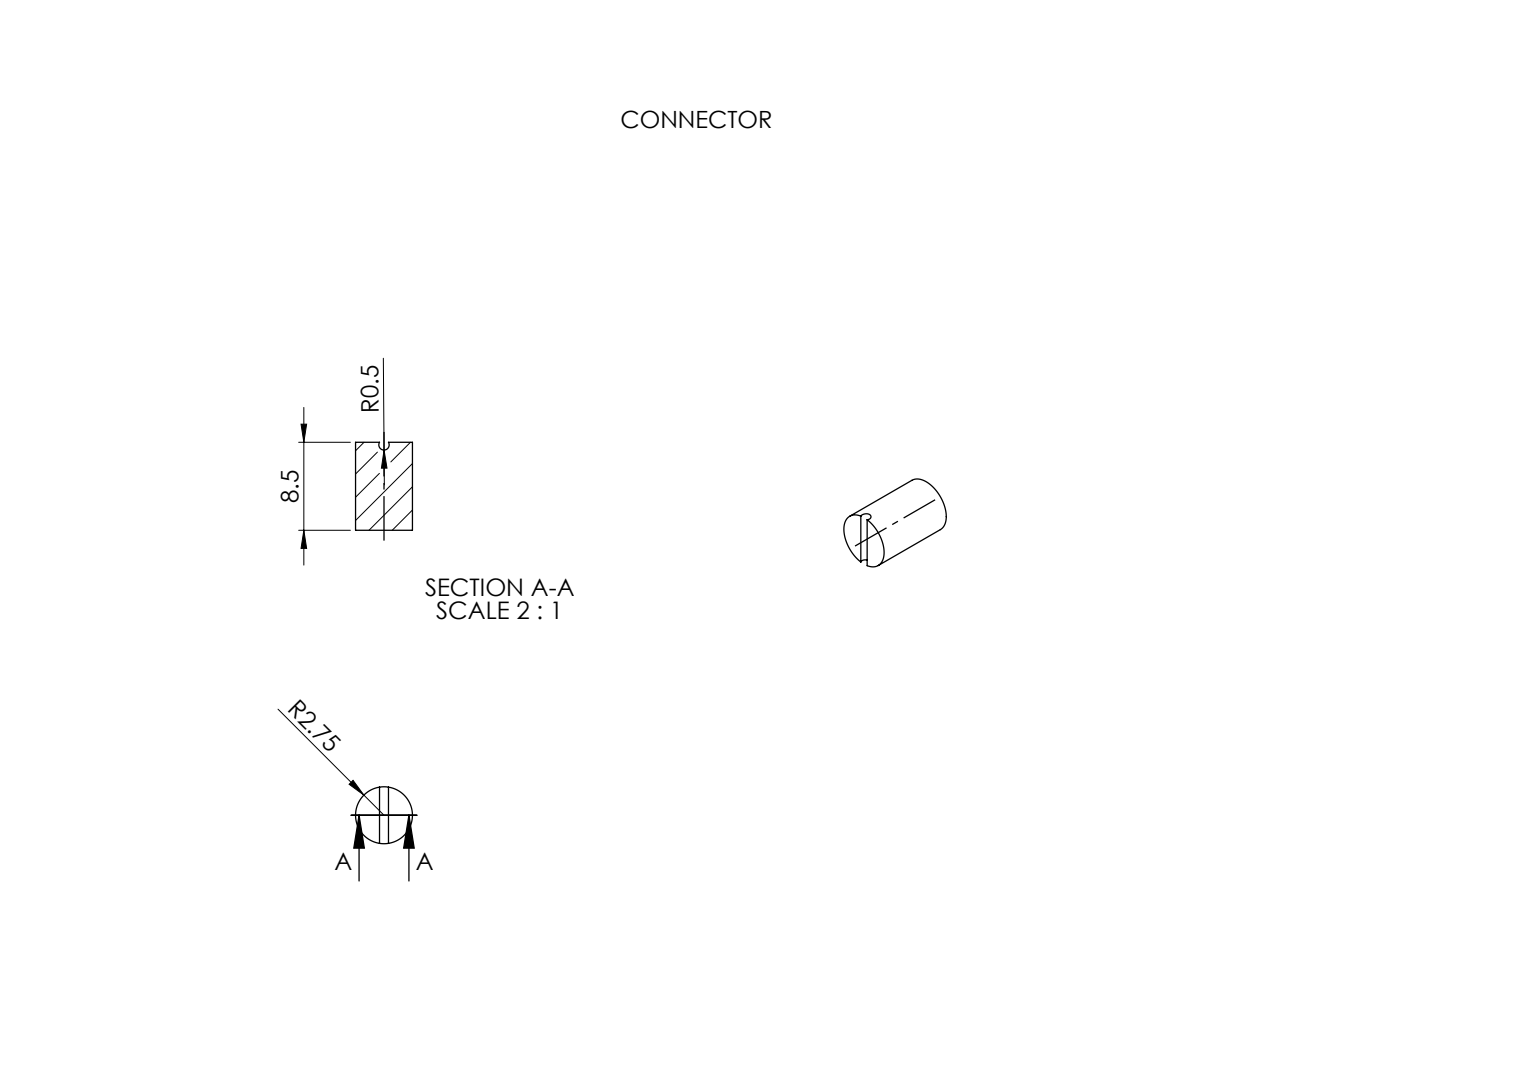
ISO-10303-21;
HEADER;
FILE_DESCRIPTION (('STEP AP214'),
    '1' );
FILE_NAME ('connector.step',
    '2026-10-05T05:16:24',
    ( '' ),
    ( '' ),
    'SwSTEP 2.0',
    'SolidWorks 2026',
    '' );
FILE_SCHEMA (( 'AUTOMOTIVE_DESIGN' ));
ENDSEC;

DATA;
#1351=DIRECTION ( 'NONE',  ( 1.000000000000000000, 0.000000000000000000, -0.000000000000000000 ) ) ;
#1835=( GEOMETRIC_REPRESENTATION_CONTEXT ( 3 ) GLOBAL_UNCERTAINTY_ASSIGNED_CONTEXT ( ( #35290 ) ) GLOBAL_UNIT_ASSIGNED_CONTEXT ( ( #39286, #45578, #18562 ) ) REPRESENTATION_CONTEXT ( 'NONE', 'WORKASPACE' ) );
#2791=VERTEX_POINT ( 'NONE', #87496 ) ;
#2984=PRODUCT_DEFINITION_FORMATION_WITH_SPECIFIED_SOURCE ( 'ANY', '', #6674, .NOT_KNOWN. ) ;
#3686=EDGE_LOOP ( 'NONE', ( #46969, #18682, #79831, #72227, #6479, #3837 ) ) ;
#3837=ORIENTED_EDGE ( 'NONE', *, *, #29448, .T. ) ;
#3884=AXIS2_PLACEMENT_3D ( 'NONE', #41339, #8443, #62915 ) ;
#3912=CARTESIAN_POINT ( 'NONE',  ( 0.4769952865663710795, -10.20868217879685425, 29.42381992869616880 ) ) ;
#4377=CARTESIAN_POINT ( 'NONE',  ( -0.1741240272142571821, -4.754468449490619086, 28.77324492963870028 ) ) ;
#4547=DIRECTION ( 'NONE',  ( -0.000000000000000000, -1.000000000000000000, -0.000000000000000000 ) ) ;
#4578=SHAPE_DEFINITION_REPRESENTATION ( #68530, #14956 ) ;
#4670=AXIS2_PLACEMENT_3D ( 'NONE', #7512, #21903, #77287 ) ;
#4814=EDGE_CURVE ( 'NONE', #33014, #88650, #15467, .T. ) ;
#5219=ADVANCED_FACE ( 'NONE', ( #76095 ), #23689, .F. ) ;
#5480=CARTESIAN_POINT ( 'NONE',  ( 1.653273178848927064E-15, -7.500000000000000000, 29.50000000000000355 ) ) ;
#5710=CARTESIAN_POINT ( 'NONE',  ( -0.4998584449498338911, -4.795810369898659609, 29.16127627612525330 ) ) ;
#6479=ORIENTED_EDGE ( 'NONE', *, *, #71103, .T. ) ;
#6620=VECTOR ( 'NONE', #30863, 1000.000000000000000 ) ;
#6674=PRODUCT ( 'connector', 'connector', '', ( #46889 ) ) ;
#7417=CARTESIAN_POINT ( 'NONE',  ( 1.653273178848927064E-15, -7.500000000000000000, 29.50000000000000355 ) ) ;
#7512=CARTESIAN_POINT ( 'NONE',  ( 1.653273178848927064E-15, -7.500000000000000000, 21.00000000000000000 ) ) ;
#8399=APPLICATION_CONTEXT ( 'automotive_design' ) ;
#8443=DIRECTION ( 'NONE',  ( -0.000000000000000000, -0.000000000000000000, -1.000000000000000000 ) ) ;
#8469=DIRECTION ( 'NONE',  ( -1.000000000000000000, 0.000000000000000000, 0.000000000000000000 ) ) ;
#9364=CARTESIAN_POINT ( 'NONE',  ( -0.08744816603778379771, -10.24999508951804650, 28.75002700765198327 ) ) ;
#9375=VERTEX_POINT ( 'NONE', #63176 ) ;
#9793=CARTESIAN_POINT ( 'NONE',  ( 0.08713905105068281420, -10.25000490179539980, 28.74997304012405408 ) ) ;
#10109=EDGE_CURVE ( 'NONE', #88311, #16692, #87365, .T. ) ;
#10152=( GEOMETRIC_REPRESENTATION_CONTEXT ( 3 ) GLOBAL_UNCERTAINTY_ASSIGNED_CONTEXT ( ( #28487 ) ) GLOBAL_UNIT_ASSIGNED_CONTEXT ( ( #73982, #12270, #74417 ) ) REPRESENTATION_CONTEXT ( 'NONE', 'WORKASPACE' ) );
#10246=CARTESIAN_POINT ( 'NONE',  ( 0.3253212748352863892, -10.23174463298371073, 28.86040964833806299 ) ) ;
#10687=CARTESIAN_POINT ( 'NONE',  ( -0.4769917816027518520, -10.20868273765699819, 29.42382599947123722 ) ) ;
#11149=DIRECTION ( 'NONE',  ( 0.000000000000000000, 0.000000000000000000, 1.000000000000000000 ) ) ;
#11285=EDGE_CURVE ( 'NONE', #16692, #40474, #43288, .T. ) ;
#12141=CARTESIAN_POINT ( 'NONE',  ( -0.4330127018922180770, -4.750000000000000000, 29.50000000000000355 ) ) ;
#12270=( NAMED_UNIT ( * ) PLANE_ANGLE_UNIT ( ) SI_UNIT ( $, .RADIAN. ) );
#13472=AXIS2_PLACEMENT_3D ( 'NONE', #74758, #27007, #74309 ) ;
#13686=EDGE_CURVE ( 'NONE', #40474, #88311, #34853, .T. ) ;
#14956=SHAPE_REPRESENTATION ( 'connector', ( #83448 ), #41778 ) ;
#14978=UNCERTAINTY_MEASURE_WITH_UNIT (LENGTH_MEASURE( 1.000000000000000082E-05 ), #26230, 'distance_accuracy_value', 'NONE');
#15253=DIRECTION ( 'NONE',  ( 1.000000000000000000, 0.000000000000000000, 0.000000000000000000 ) ) ;
#15467=CIRCLE ( 'NONE', #29797, 2.750000000000000000 ) ;
#16165=COLOUR_RGB ( '', 0.40784314, 0.44705882, 0.49803922) ;
#16692=VERTEX_POINT ( 'NONE', #79353 ) ;
#16815=EDGE_CURVE ( 'NONE', #33014, #76058, #27958, .T. ) ;
#17033=ADVANCED_BREP_SHAPE_REPRESENTATION ( '', ( #28008, #83448 ), #41778 ) ;
#17628=CARTESIAN_POINT ( 'NONE',  ( 0.4330127018922180770, -4.750000000000000000, 29.50000000000000355 ) ) ;
#17974=ORIENTED_EDGE ( 'NONE', *, *, #29448, .F. ) ;
#18120=SURFACE_SIDE_STYLE ('',( #54548 ) ) ;
#18186=ORIENTED_EDGE ( 'NONE', *, *, #10109, .T. ) ;
#18562=( NAMED_UNIT ( * ) SI_UNIT ( $, .STERADIAN. ) SOLID_ANGLE_UNIT ( ) );
#18682=ORIENTED_EDGE ( 'NONE', *, *, #62994, .F. ) ;
#18955=LINE ( 'NONE', #17628, #42535 ) ;
#19445=SURFACE_STYLE_USAGE ( .BOTH. , #18120 ) ;
#19470=SURFACE_STYLE_FILL_AREA ( #74872 ) ;
#19666=CARTESIAN_POINT ( 'NONE',  ( -0.4330127018922180770, -4.784304877199946127, 29.50000000000000355 ) ) ;
#20322=CARTESIAN_POINT ( 'NONE',  ( -2.749999999999998224, -7.500000000000000000, 29.50000000000000355 ) ) ;
#20344=EDGE_CURVE ( 'NONE', #88650, #2791, #18955, .T. ) ;
#20368=SURFACE_SIDE_STYLE ('',( #19470 ) ) ;
#21810=DIRECTION ( 'NONE',  ( 0.000000000000000000, 0.000000000000000000, 1.000000000000000000 ) ) ;
#21903=DIRECTION ( 'NONE',  ( 0.000000000000000000, 0.000000000000000000, 1.000000000000000000 ) ) ;
#22045=DIRECTION ( 'NONE',  ( 0.000000000000000000, 0.000000000000000000, 1.000000000000000000 ) ) ;
#23689=CYLINDRICAL_SURFACE ( 'NONE', #54266, 0.5000000000000004441 ) ;
#23834=CARTESIAN_POINT ( 'NONE',  ( 1.653273178848927064E-15, -7.500000000000000000, 29.50000000000000355 ) ) ;
#23893=FACE_OUTER_BOUND ( 'NONE', #86429, .T. ) ;
#24639=CARTESIAN_POINT ( 'NONE',  ( 0.3892027609374598685, -10.22267510014235370, 28.92434864502809688 ) ) ;
#24662=FACE_OUTER_BOUND ( 'NONE', #63547, .T. ) ;
#24786=AXIS2_PLACEMENT_3D ( 'NONE', #72092, #65331, #52265 ) ;
#25084=CARTESIAN_POINT ( 'NONE',  ( -0.4330127018922180770, -10.21569512280005299, 29.50000000000000355 ) ) ;
#25379=PRODUCT_DEFINITION ( 'UNKNOWN', '', #2984, #30258 ) ;
#25540=CARTESIAN_POINT ( 'NONE',  ( 0.4765651934480724106, -4.791246328801548771, 29.07531184057632601 ) ) ;
#26230=( LENGTH_UNIT ( ) NAMED_UNIT ( * ) SI_UNIT ( .MILLI., .METRE. ) );
#26433=CARTESIAN_POINT ( 'NONE',  ( -0.08713905105068302237, -4.749995098204598420, 28.74997304012405763 ) ) ;
#26982=DIRECTION ( 'NONE',  ( 0.000000000000000000, 1.000000000000000000, 0.000000000000000000 ) ) ;
#27007=DIRECTION ( 'NONE',  ( 0.000000000000000000, 0.000000000000000000, 1.000000000000000000 ) ) ;
#27623=ORIENTED_EDGE ( 'NONE', *, *, #4814, .T. ) ;
#27675=STYLED_ITEM ( 'NONE', ( #67197 ), #28008 ) ;
#27958=LINE ( 'NONE', #35154, #29073 ) ;
#28008=MANIFOLD_SOLID_BREP ( 'Cut-Extrude2', #84621 ) ;
#28487=UNCERTAINTY_MEASURE_WITH_UNIT (LENGTH_MEASURE( 1.000000000000000082E-05 ), #73982, 'distance_accuracy_value', 'NONE');
#29073=VECTOR ( 'NONE', #62180, 1000.000000000000000 ) ;
#29332=DIRECTION ( 'NONE',  ( 1.000000000000000000, 0.000000000000000000, 0.000000000000000000 ) ) ;
#29351=ORIENTED_EDGE ( 'NONE', *, *, #4814, .F. ) ;
#29448=EDGE_CURVE ( 'NONE', #9375, #76058, #45082, .T. ) ;
#29797=AXIS2_PLACEMENT_3D ( 'NONE', #7417, #21810, #83528 ) ;
#30070=CARTESIAN_POINT ( 'NONE',  ( 0.4330127018922180770, -10.21569512280005299, 29.50000000000000355 ) ) ;
#30089=DIRECTION ( 'NONE',  ( 0.000000000000000000, 0.000000000000000000, 1.000000000000000000 ) ) ;
#30129=ORIENTED_EDGE ( 'NONE', *, *, #68190, .T. ) ;
#30258=PRODUCT_DEFINITION_CONTEXT ( 'detailed design', #8399, 'design' ) ;
#30863=DIRECTION ( 'NONE',  ( -0.000000000000000000, -0.000000000000000000, -1.000000000000000000 ) ) ;
#31502=DIRECTION ( 'NONE',  ( 1.000000000000000000, 0.000000000000000000, 0.000000000000000000 ) ) ;
#31859=CARTESIAN_POINT ( 'NONE',  ( 0.3256479613346660584, -4.768304711466844203, 28.86076157308317391 ) ) ;
#32650=CARTESIAN_POINT ( 'NONE',  ( -2.749999999999998224, -7.500000000000000000, 29.50000000000000355 ) ) ;
#32990=SURFACE_STYLE_USAGE ( .BOTH. , #20368 ) ;
#33014=VERTEX_POINT ( 'NONE', #70463 ) ;
#33986=ORIENTED_EDGE ( 'NONE', *, *, #11285, .T. ) ;
#34580=FACE_OUTER_BOUND ( 'NONE', #40204, .T. ) ;
#34853=CIRCLE ( 'NONE', #85196, 2.750000000000000000 ) ;
#35154=CARTESIAN_POINT ( 'NONE',  ( 2.750000000000001776, -7.500000000000000000, 29.50000000000000355 ) ) ;
#35290=UNCERTAINTY_MEASURE_WITH_UNIT (LENGTH_MEASURE( 1.000000000000000082E-05 ), #39286, 'distance_accuracy_value', 'NONE');
#35307=DIRECTION ( 'NONE',  ( 1.000000000000000000, 0.000000000000000000, 0.000000000000000000 ) ) ;
#35668=ORIENTED_EDGE ( 'NONE', *, *, #20344, .F. ) ;
#36822=CARTESIAN_POINT ( 'NONE',  ( 0.1741240272142571821, -10.24553155050938358, 28.77324492963869673 ) ) ;
#38152=CARTESIAN_POINT ( 'NONE',  ( -0.4765651934480722995, -10.20875367119844590, 29.07531184057631890 ) ) ;
#38624=DIRECTION ( 'NONE',  ( 1.000000000000000000, 0.000000000000000000, -0.000000000000000000 ) ) ;
#38763=PLANE ( 'NONE',  #24786 ) ;
#38891=MECHANICAL_DESIGN_GEOMETRIC_PRESENTATION_REPRESENTATION('',(#48969),#10152);
#39286=( LENGTH_UNIT ( ) NAMED_UNIT ( * ) SI_UNIT ( .MILLI., .METRE. ) );
#39512=CARTESIAN_POINT ( 'NONE',  ( -0.5001402707344744236, -4.795862479435460735, 29.33712102935293231 ) ) ;
#40204=EDGE_LOOP ( 'NONE', ( #29351, #45286, #68695, #61350, #40527, #61016 ) ) ;
#40398=CARTESIAN_POINT ( 'NONE',  ( 0.3891064303782384992, -4.777307027835201225, 28.92407589458995432 ) ) ;
#40474=VERTEX_POINT ( 'NONE', #20322 ) ;
#40527=ORIENTED_EDGE ( 'NONE', *, *, #11285, .F. ) ;
#41339=CARTESIAN_POINT ( 'NONE',  ( 1.653273178848927064E-15, -7.500000000000000000, 29.50000000000000355 ) ) ;
#41751=B_SPLINE_CURVE_WITH_KNOTS ( 'NONE', 3,
 ( #52111, #79600, #87260, #87707, #25540, #40398, #31859, #80040, #75067, #26433, #4377, #67856, #66066, #73744, #5710, #39512, #46254, #19666 ),
 .UNSPECIFIED., .F., .F.,
 ( 4, 2, 2, 2, 2, 2, 2, 2, 4 ),
 ( 0.000000000000000000, 0.0002610006692907291767, 0.0005220013385814583533, 0.0007830020078721875842, 0.001044002677162916707, 0.001305003346453645829, 0.001566004015744375168, 0.001827004685035104291, 0.002088005354325833413 ),
 .UNSPECIFIED. ) ;
#41778=( GEOMETRIC_REPRESENTATION_CONTEXT ( 3 ) GLOBAL_UNCERTAINTY_ASSIGNED_CONTEXT ( ( #14978 ) ) GLOBAL_UNIT_ASSIGNED_CONTEXT ( ( #26230, #60453, #87970 ) ) REPRESENTATION_CONTEXT ( 'NONE', 'WORKASPACE' ) );
#41884=CARTESIAN_POINT ( 'NONE',  ( 0.000000000000000000, -4.750000000000000000, 29.25000000000000000 ) ) ;
#42535=VECTOR ( 'NONE', #4547, 1000.000000000000000 ) ;
#42552=EDGE_CURVE ( 'NONE', #88650, #16692, #41751, .T. ) ;
#43038=ORIENTED_EDGE ( 'NONE', *, *, #55374, .F. ) ;
#43288=CIRCLE ( 'NONE', #79214, 2.750000000000000000 ) ;
#44818=LINE ( 'NONE', #32650, #6620 ) ;
#45082=CIRCLE ( 'NONE', #13472, 2.750000000000000000 ) ;
#45286=ORIENTED_EDGE ( 'NONE', *, *, #16815, .T. ) ;
#45346=CARTESIAN_POINT ( 'NONE',  ( -0.3891064303782384992, -10.22269297216479877, 28.92407589458995432 ) ) ;
#45578=( NAMED_UNIT ( * ) PLANE_ANGLE_UNIT ( ) SI_UNIT ( $, .RADIAN. ) );
#46254=CARTESIAN_POINT ( 'NONE',  ( -0.4769952865663709130, -4.791317821203144867, 29.42381992869616880 ) ) ;
#46889=PRODUCT_CONTEXT ( 'NONE', #82604, 'mechanical' ) ;
#46969=ORIENTED_EDGE ( 'NONE', *, *, #16815, .F. ) ;
#47379=SHAPE_REPRESENTATION_RELATIONSHIP ( 'NONE' , 'NONE' ,  #14956, #17033 ) ;
#48107=CYLINDRICAL_SURFACE ( 'NONE', #79255, 2.750000000000000000 ) ;
#48969=STYLED_ITEM ( 'NONE', ( #88841 ), #17033 ) ;
#50513=ORIENTED_EDGE ( 'NONE', *, *, #20344, .T. ) ;
#51640=CARTESIAN_POINT ( 'NONE',  ( -0.1752029071980582831, -10.24545254656222149, 28.77370482994317058 ) ) ;
#52111=CARTESIAN_POINT ( 'NONE',  ( 0.4330127018922180770, -4.784304877199946127, 29.50000000000000355 ) ) ;
#52126=PLANE ( 'NONE',  #54565 ) ;
#52265=DIRECTION ( 'NONE',  ( 1.000000000000000000, 0.000000000000000000, -0.000000000000000000 ) ) ;
#53068=ADVANCED_FACE ( 'NONE', ( #83695 ), #48107, .T. ) ;
#53177=ORIENTED_EDGE ( 'NONE', *, *, #62994, .T. ) ;
#53488=EDGE_LOOP ( 'NONE', ( #30129, #35668, #71447, #76985 ) ) ;
#53522=CIRCLE ( 'NONE', #4670, 2.750000000000000000 ) ;
#54266=AXIS2_PLACEMENT_3D ( 'NONE', #41884, #69786, #22045 ) ;
#54548=SURFACE_STYLE_FILL_AREA ( #61299 ) ;
#54565=AXIS2_PLACEMENT_3D ( 'NONE', #79614, #11149, #38624 ) ;
#55374=EDGE_CURVE ( 'NONE', #76058, #9375, #53522, .T. ) ;
#55410=CARTESIAN_POINT ( 'NONE',  ( 1.653273178848927064E-15, -7.500000000000000000, 29.50000000000000355 ) ) ;
#57551=ADVANCED_FACE ( 'NONE', ( #23893 ), #38763, .F. ) ;
#57975=CARTESIAN_POINT ( 'NONE',  ( -0.5000075107691263065, -10.20416206785629498, 29.33696104038924446 ) ) ;
#59725=CARTESIAN_POINT ( 'NONE',  ( 2.750000000000001776, -7.500000000000000000, 21.00000000000000000 ) ) ;
#60453=( NAMED_UNIT ( * ) PLANE_ANGLE_UNIT ( ) SI_UNIT ( $, .RADIAN. ) );
#61016=ORIENTED_EDGE ( 'NONE', *, *, #42552, .F. ) ;
#61299=FILL_AREA_STYLE ('',( #81160 ) ) ;
#61350=ORIENTED_EDGE ( 'NONE', *, *, #71103, .F. ) ;
#61893=COLOUR_RGB ( '', 0.40784314, 0.44705882, 0.49803922) ;
#62180=DIRECTION ( 'NONE',  ( -0.000000000000000000, -0.000000000000000000, -1.000000000000000000 ) ) ;
#62206=MECHANICAL_DESIGN_GEOMETRIC_PRESENTATION_REPRESENTATION('',(#27675),#1835);
#62763=CARTESIAN_POINT ( 'NONE',  ( 0.000000000000000000, 0.000000000000000000, 0.000000000000000000 ) ) ;
#62915=DIRECTION ( 'NONE',  ( -1.000000000000000000, 0.000000000000000000, 0.000000000000000000 ) ) ;
#62994=EDGE_CURVE ( 'NONE', #2791, #33014, #70001, .T. ) ;
#63176=CARTESIAN_POINT ( 'NONE',  ( -2.749999999999998224, -7.500000000000000000, 21.00000000000000000 ) ) ;
#63542=DIRECTION ( 'NONE',  ( 0.000000000000000000, 0.000000000000000000, 1.000000000000000000 ) ) ;
#63547=EDGE_LOOP ( 'NONE', ( #33986, #76979, #18186 ) ) ;
#64723=CARTESIAN_POINT ( 'NONE',  ( 0.4761625575576028391, -10.20882035374011565, 29.07450979259063928 ) ) ;
#65031=EDGE_LOOP ( 'NONE', ( #53177, #27623, #50513 ) ) ;
#65331=DIRECTION ( 'NONE',  ( 0.000000000000000000, 0.000000000000000000, 1.000000000000000000 ) ) ;
#66059=CARTESIAN_POINT ( 'NONE',  ( 0.5001402707344744236, -10.20413752056454193, 29.33712102935293942 ) ) ;
#66066=CARTESIAN_POINT ( 'NONE',  ( -0.3892027609374598685, -4.777324899857646301, 28.92434864502810399 ) ) ;
#66807=ADVANCED_FACE ( 'NONE', ( #77021 ), #70257, .T. ) ;
#67197=PRESENTATION_STYLE_ASSIGNMENT (( #19445 ) ) ;
#67856=CARTESIAN_POINT ( 'NONE',  ( -0.3253212748352862782, -4.768255367016290158, 28.86040964833806299 ) ) ;
#68190=EDGE_CURVE ( 'NONE', #88311, #2791, #83175, .T. ) ;
#68530=PRODUCT_DEFINITION_SHAPE ( 'NONE', 'NONE',  #25379 ) ;
#68695=ORIENTED_EDGE ( 'NONE', *, *, #55374, .T. ) ;
#69786=DIRECTION ( 'NONE',  ( 0.000000000000000000, 1.000000000000000000, 0.000000000000000000 ) ) ;
#69812=DIRECTION ( 'NONE',  ( 0.000000000000000000, 0.000000000000000000, 1.000000000000000000 ) ) ;
#70001=CIRCLE ( 'NONE', #78617, 2.750000000000000000 ) ;
#70158=DIRECTION ( 'NONE',  ( -0.000000000000000000, -0.000000000000000000, -1.000000000000000000 ) ) ;
#70257=PLANE ( 'NONE',  #73946 ) ;
#70463=CARTESIAN_POINT ( 'NONE',  ( 2.750000000000001776, -7.500000000000000000, 29.50000000000000355 ) ) ;
#70474=VECTOR ( 'NONE', #26982, 1000.000000000000000 ) ;
#71050=CARTESIAN_POINT ( 'NONE',  ( -0.4999924855028897164, -10.20416484602898954, 29.16295261168903252 ) ) ;
#71103=EDGE_CURVE ( 'NONE', #40474, #9375, #44818, .T. ) ;
#71447=ORIENTED_EDGE ( 'NONE', *, *, #42552, .T. ) ;
#71935=CARTESIAN_POINT ( 'NONE',  ( -0.3256479613346683899, -10.23169528853315491, 28.86076157308317391 ) ) ;
#72092=CARTESIAN_POINT ( 'NONE',  ( 1.653273178848927064E-15, -7.500000000000000000, 21.00000000000000000 ) ) ;
#72227=ORIENTED_EDGE ( 'NONE', *, *, #13686, .F. ) ;
#73744=CARTESIAN_POINT ( 'NONE',  ( -0.4761625575576027836, -4.791179646259885239, 29.07450979259064638 ) ) ;
#73946=AXIS2_PLACEMENT_3D ( 'NONE', #55410, #69812, #1351 ) ;
#73982=( LENGTH_UNIT ( ) NAMED_UNIT ( * ) SI_UNIT ( .MILLI., .METRE. ) );
#74309=DIRECTION ( 'NONE',  ( 1.000000000000000000, 0.000000000000000000, 0.000000000000000000 ) ) ;
#74417=( NAMED_UNIT ( * ) SI_UNIT ( $, .STERADIAN. ) SOLID_ANGLE_UNIT ( ) );
#74758=CARTESIAN_POINT ( 'NONE',  ( 1.653273178848927064E-15, -7.500000000000000000, 21.00000000000000000 ) ) ;
#74872=FILL_AREA_STYLE ('',( #81624 ) ) ;
#75067=CARTESIAN_POINT ( 'NONE',  ( 0.08744816603778360342, -4.750004910481952614, 28.75002700765199037 ) ) ;
#75557=CYLINDRICAL_SURFACE ( 'NONE', #3884, 2.750000000000000000 ) ;
#75889=ADVANCED_FACE ( 'NONE', ( #34580 ), #75557, .T. ) ;
#76058=VERTEX_POINT ( 'NONE', #59725 ) ;
#76095=FACE_OUTER_BOUND ( 'NONE', #53488, .T. ) ;
#76949=CARTESIAN_POINT ( 'NONE',  ( 1.653273178848927064E-15, -7.500000000000000000, 29.50000000000000355 ) ) ;
#76979=ORIENTED_EDGE ( 'NONE', *, *, #13686, .T. ) ;
#76985=ORIENTED_EDGE ( 'NONE', *, *, #10109, .F. ) ;
#77021=FACE_OUTER_BOUND ( 'NONE', #65031, .T. ) ;
#77287=DIRECTION ( 'NONE',  ( 1.000000000000000000, 0.000000000000000000, 0.000000000000000000 ) ) ;
#77948=CARTESIAN_POINT ( 'NONE',  ( 1.653273178848927064E-15, -7.500000000000000000, 29.50000000000000355 ) ) ;
#78617=AXIS2_PLACEMENT_3D ( 'NONE', #23834, #86006, #31502 ) ;
#79214=AXIS2_PLACEMENT_3D ( 'NONE', #76949, #30089, #15253 ) ;
#79255=AXIS2_PLACEMENT_3D ( 'NONE', #5480, #70158, #8469 ) ;
#79353=CARTESIAN_POINT ( 'NONE',  ( -0.4330127018922180770, -4.784304877199946127, 29.50000000000000355 ) ) ;
#79600=CARTESIAN_POINT ( 'NONE',  ( 0.4769917816027516855, -4.791317262343001815, 29.42382599947123722 ) ) ;
#79614=CARTESIAN_POINT ( 'NONE',  ( 1.653273178848927064E-15, -7.500000000000000000, 29.50000000000000355 ) ) ;
#79831=ORIENTED_EDGE ( 'NONE', *, *, #68190, .F. ) ;
#80040=CARTESIAN_POINT ( 'NONE',  ( 0.1752029071980549801, -4.754547453437774074, 28.77370482994318124 ) ) ;
#81160=FILL_AREA_STYLE_COLOUR ( '', #16165 ) ;
#81624=FILL_AREA_STYLE_COLOUR ( '', #61893 ) ;
#82604=APPLICATION_CONTEXT ( 'automotive_design' ) ;
#83175=B_SPLINE_CURVE_WITH_KNOTS ( 'NONE', 3,
 ( #25084, #10687, #57975, #71050, #38152, #45346, #71935, #51640, #9364, #9793, #36822, #10246, #24639, #64723, #85902, #66059, #3912, #30070 ),
 .UNSPECIFIED., .F., .F.,
 ( 4, 2, 2, 2, 2, 2, 2, 2, 4 ),
 ( 0.000000000000000000, 0.0002610006692907291224, 0.0005220013385814582449, 0.0007830020078721873673, 0.001044002677162916490, 0.001305003346453645612, 0.001566004015744375168, 0.001827004685035104291, 0.002088005354325833847 ),
 .UNSPECIFIED. ) ;
#83448=AXIS2_PLACEMENT_3D ( 'NONE', #62763, #83959, #35307 ) ;
#83528=DIRECTION ( 'NONE',  ( 1.000000000000000000, 0.000000000000000000, 0.000000000000000000 ) ) ;
#83695=FACE_OUTER_BOUND ( 'NONE', #3686, .T. ) ;
#83959=DIRECTION ( 'NONE',  ( 0.000000000000000000, 0.000000000000000000, 1.000000000000000000 ) ) ;
#84382=CARTESIAN_POINT ( 'NONE',  ( -0.4330127018922180770, -10.21569512280005299, 29.50000000000000355 ) ) ;
#84621=CLOSED_SHELL ( 'NONE', ( #75889, #53068, #66807, #88763, #57551, #5219 ) ) ;
#85196=AXIS2_PLACEMENT_3D ( 'NONE', #77948, #63542, #29332 ) ;
#85902=CARTESIAN_POINT ( 'NONE',  ( 0.4998584449498339466, -10.20418963010134306, 29.16127627612525330 ) ) ;
#86006=DIRECTION ( 'NONE',  ( 0.000000000000000000, 0.000000000000000000, 1.000000000000000000 ) ) ;
#86429=EDGE_LOOP ( 'NONE', ( #17974, #43038 ) ) ;
#87260=CARTESIAN_POINT ( 'NONE',  ( 0.5000075107691263065, -4.795837932143704130, 29.33696104038925156 ) ) ;
#87365=LINE ( 'NONE', #12141, #70474 ) ;
#87496=CARTESIAN_POINT ( 'NONE',  ( 0.4330127018922180770, -10.21569512280005299, 29.50000000000000355 ) ) ;
#87707=CARTESIAN_POINT ( 'NONE',  ( 0.4999924855028897164, -4.795835153971004239, 29.16295261168902542 ) ) ;
#87725=CARTESIAN_POINT ( 'NONE',  ( 0.4330127018922180770, -4.784304877199946127, 29.50000000000000355 ) ) ;
#87970=( NAMED_UNIT ( * ) SI_UNIT ( $, .STERADIAN. ) SOLID_ANGLE_UNIT ( ) );
#88311=VERTEX_POINT ( 'NONE', #84382 ) ;
#88650=VERTEX_POINT ( 'NONE', #87725 ) ;
#88763=ADVANCED_FACE ( 'NONE', ( #24662 ), #52126, .T. ) ;
#88841=PRESENTATION_STYLE_ASSIGNMENT (( #32990 ) ) ;
ENDSEC;
END-ISO-10303-21;
